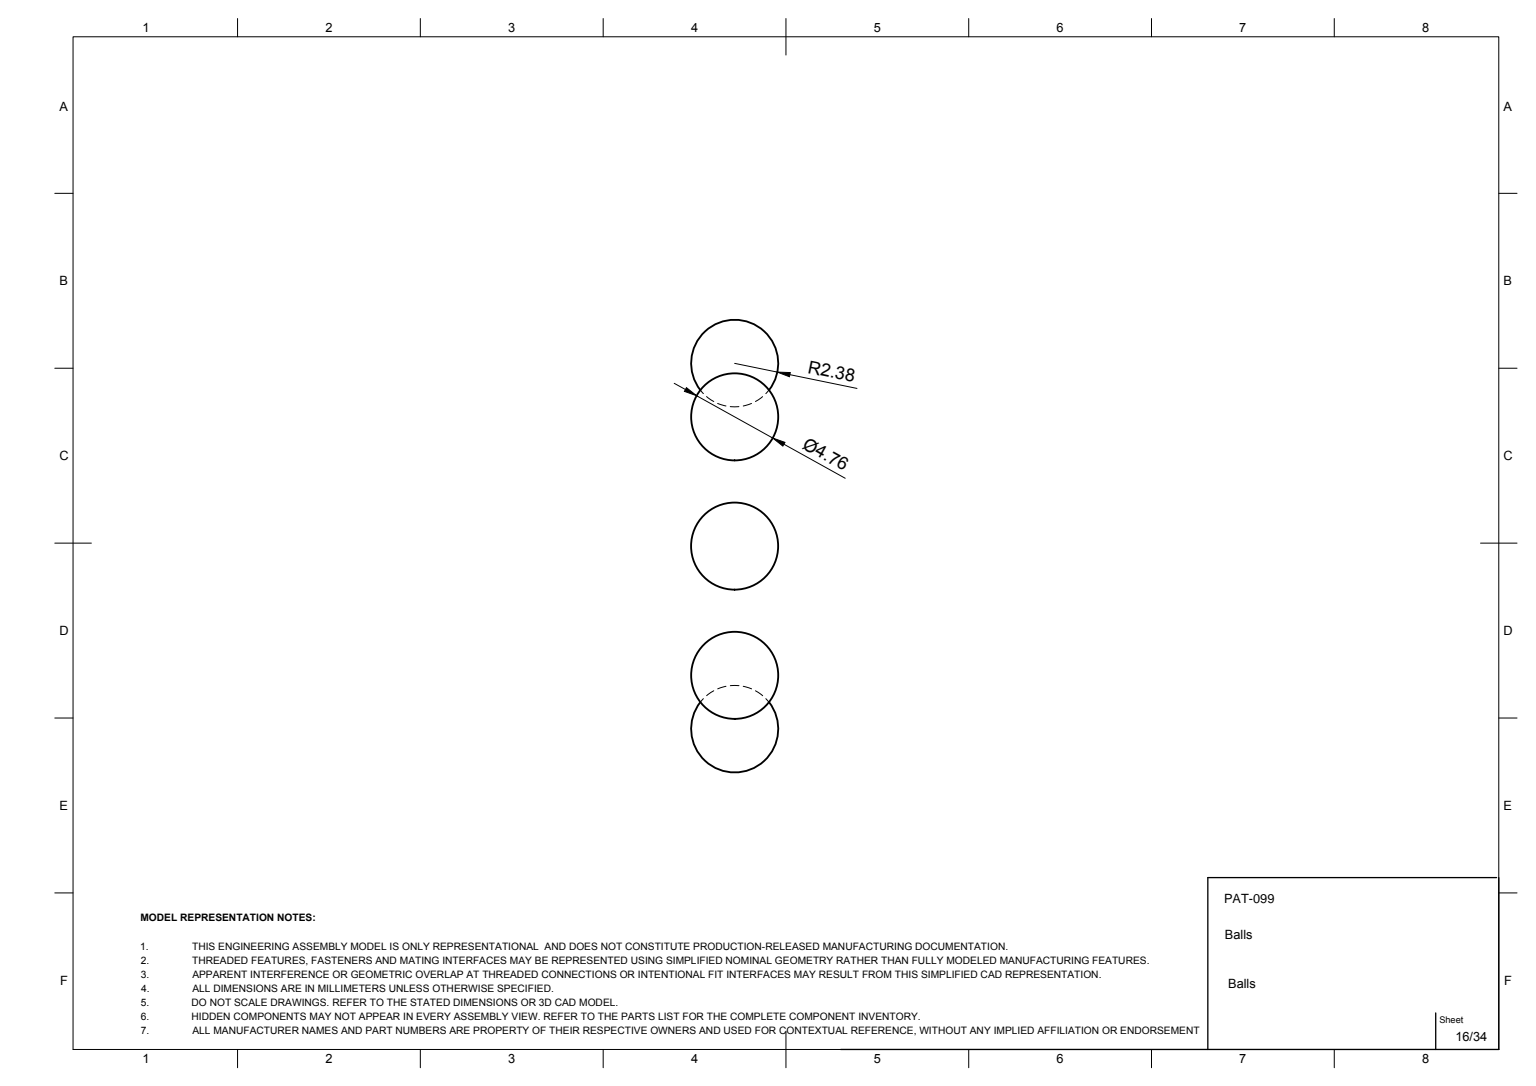
ISO-10303-21;
HEADER;
/* Generated by software containing ST-Developer
 * from STEP Tools, Inc. (www.steptools.com) 
 */

FILE_DESCRIPTION(
/* description */ ('PAT-099'),
/* implementation_level */ '2;1');

FILE_NAME(
/* name */ 'Balls.step',
/* time_stamp */ '2026-10-29T17:25:42-07:00',
/* author */ (''),
/* organization */ (''),
/* preprocessor_version */ 'ST-DEVELOPER v20.2',
/* originating_system */ 'Autodesk Translation Framework v15.17.0.0',
/* authorisation */ '');

FILE_SCHEMA (('AUTOMOTIVE_DESIGN { 1 0 10303 214 3 1 1 }'));
ENDSEC;

DATA;
#10=MECHANICAL_DESIGN_GEOMETRIC_PRESENTATION_REPRESENTATION('',(#359,#360,#361,#362,#363,#364,#365,#366),#11035);
#11=SPHERICAL_SURFACE('',#5544,0.23815);
#12=SPHERICAL_SURFACE('',#5546,0.23815);
#13=SPHERICAL_SURFACE('',#5548,0.23815);
#14=SPHERICAL_SURFACE('',#5550,0.23815);
#15=SPHERICAL_SURFACE('',#5552,0.23815);
#16=SPHERICAL_SURFACE('',#5554,0.23815);
#17=SPHERICAL_SURFACE('',#5556,0.23815);
#18=SPHERICAL_SURFACE('',#5558,0.23815);
#309=SHAPE_REPRESENTATION_RELATIONSHIP('SRR','None',#11182,#334);
#334=ADVANCED_BREP_SHAPE_REPRESENTATION('',(#390,#391,#392,#393,#394,#395,
#396,#397),#11032);
#359=STYLED_ITEM('',(#11386),#390);
#360=STYLED_ITEM('',(#11386),#391);
#361=STYLED_ITEM('',(#11386),#392);
#362=STYLED_ITEM('',(#11386),#393);
#363=STYLED_ITEM('',(#11386),#394);
#364=STYLED_ITEM('',(#11386),#395);
#365=STYLED_ITEM('',(#11386),#396);
#366=STYLED_ITEM('',(#11386),#397);
#390=MANIFOLD_SOLID_BREP('Body1',#4729);
#391=MANIFOLD_SOLID_BREP('Body2',#4730);
#392=MANIFOLD_SOLID_BREP('Body3',#4731);
#393=MANIFOLD_SOLID_BREP('Body4',#4732);
#394=MANIFOLD_SOLID_BREP('Body5',#4733);
#395=MANIFOLD_SOLID_BREP('Body6',#4734);
#396=MANIFOLD_SOLID_BREP('Body7',#4735);
#397=MANIFOLD_SOLID_BREP('Body8',#4736);
#905=FACE_OUTER_BOUND('',#1303,.T.);
#906=FACE_OUTER_BOUND('',#1304,.T.);
#907=FACE_OUTER_BOUND('',#1305,.T.);
#908=FACE_OUTER_BOUND('',#1306,.T.);
#909=FACE_OUTER_BOUND('',#1307,.T.);
#910=FACE_OUTER_BOUND('',#1308,.T.);
#911=FACE_OUTER_BOUND('',#1309,.T.);
#912=FACE_OUTER_BOUND('',#1310,.T.);
#1303=EDGE_LOOP('',(#4161,#4162));
#1304=EDGE_LOOP('',(#4163,#4164));
#1305=EDGE_LOOP('',(#4165,#4166));
#1306=EDGE_LOOP('',(#4167,#4168));
#1307=EDGE_LOOP('',(#4169,#4170));
#1308=EDGE_LOOP('',(#4171,#4172));
#1309=EDGE_LOOP('',(#4173,#4174));
#1310=EDGE_LOOP('',(#4175,#4176));
#2088=CIRCLE('',#5545,0.23815);
#2089=CIRCLE('',#5547,0.23815);
#2090=CIRCLE('',#5549,0.23815);
#2091=CIRCLE('',#5551,0.23815);
#2092=CIRCLE('',#5553,0.23815);
#2093=CIRCLE('',#5555,0.23815);
#2094=CIRCLE('',#5557,0.23815);
#2095=CIRCLE('',#5559,0.23815);
#2482=VERTEX_POINT('',#10425);
#2483=VERTEX_POINT('',#10426);
#2484=VERTEX_POINT('',#10429);
#2485=VERTEX_POINT('',#10430);
#2486=VERTEX_POINT('',#10433);
#2487=VERTEX_POINT('',#10434);
#2488=VERTEX_POINT('',#10437);
#2489=VERTEX_POINT('',#10438);
#2490=VERTEX_POINT('',#10441);
#2491=VERTEX_POINT('',#10442);
#2492=VERTEX_POINT('',#10445);
#2493=VERTEX_POINT('',#10446);
#2494=VERTEX_POINT('',#10449);
#2495=VERTEX_POINT('',#10450);
#2496=VERTEX_POINT('',#10453);
#2497=VERTEX_POINT('',#10454);
#3057=EDGE_CURVE('',#2482,#2483,#2088,.T.);
#3058=EDGE_CURVE('',#2484,#2485,#2089,.T.);
#3059=EDGE_CURVE('',#2486,#2487,#2090,.T.);
#3060=EDGE_CURVE('',#2488,#2489,#2091,.T.);
#3061=EDGE_CURVE('',#2490,#2491,#2092,.T.);
#3062=EDGE_CURVE('',#2492,#2493,#2093,.T.);
#3063=EDGE_CURVE('',#2494,#2495,#2094,.T.);
#3064=EDGE_CURVE('',#2496,#2497,#2095,.T.);
#4161=ORIENTED_EDGE('',*,*,#3057,.T.);
#4162=ORIENTED_EDGE('',*,*,#3057,.F.);
#4163=ORIENTED_EDGE('',*,*,#3058,.T.);
#4164=ORIENTED_EDGE('',*,*,#3058,.F.);
#4165=ORIENTED_EDGE('',*,*,#3059,.T.);
#4166=ORIENTED_EDGE('',*,*,#3059,.F.);
#4167=ORIENTED_EDGE('',*,*,#3060,.T.);
#4168=ORIENTED_EDGE('',*,*,#3060,.F.);
#4169=ORIENTED_EDGE('',*,*,#3061,.T.);
#4170=ORIENTED_EDGE('',*,*,#3061,.F.);
#4171=ORIENTED_EDGE('',*,*,#3062,.T.);
#4172=ORIENTED_EDGE('',*,*,#3062,.F.);
#4173=ORIENTED_EDGE('',*,*,#3063,.T.);
#4174=ORIENTED_EDGE('',*,*,#3063,.F.);
#4175=ORIENTED_EDGE('',*,*,#3064,.T.);
#4176=ORIENTED_EDGE('',*,*,#3064,.F.);
#4670=ADVANCED_FACE('',(#905),#11,.T.);
#4671=ADVANCED_FACE('',(#906),#12,.T.);
#4672=ADVANCED_FACE('',(#907),#13,.T.);
#4673=ADVANCED_FACE('',(#908),#14,.T.);
#4674=ADVANCED_FACE('',(#909),#15,.T.);
#4675=ADVANCED_FACE('',(#910),#16,.T.);
#4676=ADVANCED_FACE('',(#911),#17,.T.);
#4677=ADVANCED_FACE('',(#912),#18,.T.);
#4729=CLOSED_SHELL('',(#4670));
#4730=CLOSED_SHELL('',(#4671));
#4731=CLOSED_SHELL('',(#4672));
#4732=CLOSED_SHELL('',(#4673));
#4733=CLOSED_SHELL('',(#4674));
#4734=CLOSED_SHELL('',(#4675));
#4735=CLOSED_SHELL('',(#4676));
#4736=CLOSED_SHELL('',(#4677));
#5543=AXIS2_PLACEMENT_3D('',#10423,#6968,#6969);
#5544=AXIS2_PLACEMENT_3D('',#10424,#6970,#6971);
#5545=AXIS2_PLACEMENT_3D('',#10427,#6972,#6973);
#5546=AXIS2_PLACEMENT_3D('',#10428,#6974,#6975);
#5547=AXIS2_PLACEMENT_3D('',#10431,#6976,#6977);
#5548=AXIS2_PLACEMENT_3D('',#10432,#6978,#6979);
#5549=AXIS2_PLACEMENT_3D('',#10435,#6980,#6981);
#5550=AXIS2_PLACEMENT_3D('',#10436,#6982,#6983);
#5551=AXIS2_PLACEMENT_3D('',#10439,#6984,#6985);
#5552=AXIS2_PLACEMENT_3D('',#10440,#6986,#6987);
#5553=AXIS2_PLACEMENT_3D('',#10443,#6988,#6989);
#5554=AXIS2_PLACEMENT_3D('',#10444,#6990,#6991);
#5555=AXIS2_PLACEMENT_3D('',#10447,#6992,#6993);
#5556=AXIS2_PLACEMENT_3D('',#10448,#6994,#6995);
#5557=AXIS2_PLACEMENT_3D('',#10451,#6996,#6997);
#5558=AXIS2_PLACEMENT_3D('',#10452,#6998,#6999);
#5559=AXIS2_PLACEMENT_3D('',#10455,#7000,#7001);
#6968=DIRECTION('axis',(0.,0.,1.));
#6969=DIRECTION('refdir',(1.,0.,0.));
#6970=DIRECTION('center_axis',(0.,0.,1.));
#6971=DIRECTION('ref_axis',(1.,0.,0.));
#6972=DIRECTION('center_axis',(1.22464679914735E-16,-1.,0.));
#6973=DIRECTION('ref_axis',(-1.,-1.22464679914735E-16,0.));
#6974=DIRECTION('center_axis',(0.707106781186548,0.,0.707106781186548));
#6975=DIRECTION('ref_axis',(0.707106781186548,0.,-0.707106781186548));
#6976=DIRECTION('center_axis',(8.65956056235494E-17,-1.,-8.65956056235493E-17));
#6977=DIRECTION('ref_axis',(-0.707106781186547,-1.22464679914735E-16,0.707106781186547));
#6978=DIRECTION('center_axis',(1.,0.,0.));
#6979=DIRECTION('ref_axis',(6.12323399573676E-17,0.,-1.));
#6980=DIRECTION('center_axis',(7.49879891330929E-33,-1.,-1.22464679914735E-16));
#6981=DIRECTION('ref_axis',(-6.12323399573676E-17,-1.22464679914735E-16,
1.));
#6982=DIRECTION('center_axis',(0.707106781186548,0.,-0.707106781186548));
#6983=DIRECTION('ref_axis',(-0.707106781186548,0.,-0.707106781186548));
#6984=DIRECTION('center_axis',(-8.65956056235493E-17,-1.,-8.65956056235494E-17));
#6985=DIRECTION('ref_axis',(0.707106781186547,-1.22464679914735E-16,0.707106781186547));
#6986=DIRECTION('center_axis',(0.,0.,-1.));
#6987=DIRECTION('ref_axis',(-1.,0.,-1.22464679914735E-16));
#6988=DIRECTION('center_axis',(-1.22464679914735E-16,-1.,-1.49975978266186E-32));
#6989=DIRECTION('ref_axis',(1.,-1.22464679914735E-16,1.22464679914735E-16));
#6990=DIRECTION('center_axis',(-0.707106781186547,0.,-0.707106781186548));
#6991=DIRECTION('ref_axis',(-0.707106781186548,0.,0.707106781186547));
#6992=DIRECTION('center_axis',(-8.65956056235493E-17,-1.,8.65956056235493E-17));
#6993=DIRECTION('ref_axis',(0.707106781186548,-1.22464679914735E-16,-0.707106781186547));
#6994=DIRECTION('center_axis',(-1.,0.,0.));
#6995=DIRECTION('ref_axis',(-1.83697019872103E-16,0.,1.));
#6996=DIRECTION('center_axis',(-2.24963967399279E-32,-1.,1.22464679914735E-16));
#6997=DIRECTION('ref_axis',(1.83697019872103E-16,-1.22464679914735E-16,
-1.));
#6998=DIRECTION('center_axis',(-0.707106781186548,0.,0.707106781186548));
#6999=DIRECTION('ref_axis',(0.707106781186547,0.,0.707106781186548));
#7000=DIRECTION('center_axis',(8.65956056235493E-17,-1.,8.65956056235493E-17));
#7001=DIRECTION('ref_axis',(-0.707106781186547,-1.22464679914735E-16,-0.707106781186548));
#10423=CARTESIAN_POINT('',(0.,0.,0.));
#10424=CARTESIAN_POINT('Origin',(1.,0.,0.));
#10425=CARTESIAN_POINT('',(1.,-1.78583896120461E-33,0.23815));
#10426=CARTESIAN_POINT('',(1.,-1.78583896120461E-33,-0.23815));
#10427=CARTESIAN_POINT('Origin',(1.,0.,0.));
#10428=CARTESIAN_POINT('Origin',(0.707106781186548,0.,-0.707106781186547));
#10429=CARTESIAN_POINT('',(0.875504261126124,-1.78583896120461E-33,-0.538709301246971));
#10430=CARTESIAN_POINT('',(0.538709301246971,-1.78583896120461E-33,-0.875504261126124));
#10431=CARTESIAN_POINT('Origin',(0.707106781186548,0.,-0.707106781186547));
#10432=CARTESIAN_POINT('Origin',(6.12323399573677E-17,0.,-1.));
#10433=CARTESIAN_POINT('',(0.23815,-1.78583896120461E-33,-1.));
#10434=CARTESIAN_POINT('',(-0.23815,-1.78583896120461E-33,-1.));
#10435=CARTESIAN_POINT('Origin',(6.12323399573677E-17,0.,-1.));
#10436=CARTESIAN_POINT('Origin',(-0.707106781186547,0.,-0.707106781186548));
#10437=CARTESIAN_POINT('',(-0.538709301246971,-1.78583896120461E-33,-0.875504261126124));
#10438=CARTESIAN_POINT('',(-0.875504261126124,-1.78583896120461E-33,-0.538709301246971));
#10439=CARTESIAN_POINT('Origin',(-0.707106781186547,0.,-0.707106781186548));
#10440=CARTESIAN_POINT('Origin',(-1.,0.,-1.22464679914735E-16));
#10441=CARTESIAN_POINT('',(-1.,-1.78583896120461E-33,-0.23815));
#10442=CARTESIAN_POINT('',(-1.,-1.78583896120461E-33,0.23815));
#10443=CARTESIAN_POINT('Origin',(-1.,0.,-1.22464679914735E-16));
#10444=CARTESIAN_POINT('Origin',(-0.707106781186548,0.,0.707106781186547));
#10445=CARTESIAN_POINT('',(-0.875504261126124,-7.94881478324376E-33,0.538709301246971));
#10446=CARTESIAN_POINT('',(-0.538709301246971,4.37713686083455E-33,0.875504261126124));
#10447=CARTESIAN_POINT('Origin',(-0.707106781186548,0.,0.707106781186547));
#10448=CARTESIAN_POINT('Origin',(-1.83697019872103E-16,0.,1.));
#10449=CARTESIAN_POINT('',(-0.23815,-1.78583896120461E-33,1.));
#10450=CARTESIAN_POINT('',(0.23815,-1.78583896120461E-33,1.));
#10451=CARTESIAN_POINT('Origin',(-1.83697019872103E-16,0.,1.));
#10452=CARTESIAN_POINT('Origin',(0.707106781186547,0.,0.707106781186548));
#10453=CARTESIAN_POINT('',(0.538709301246971,-4.86732687222419E-33,0.875504261126124));
#10454=CARTESIAN_POINT('',(0.875504261126124,1.29564894981497E-33,0.538709301246971));
#10455=CARTESIAN_POINT('Origin',(0.707106781186547,0.,0.707106781186548));
#10999=UNCERTAINTY_MEASURE_WITH_UNIT(LENGTH_MEASURE(0.001),#11036,
'DISTANCE_ACCURACY_VALUE',
'Maximum model space distance between geometric entities at asserted c
onnectivities');
#11002=UNCERTAINTY_MEASURE_WITH_UNIT(LENGTH_MEASURE(0.001),#11036,
'DISTANCE_ACCURACY_VALUE',
'Maximum model space distance between geometric entities at asserted c
onnectivities');
#11032=(
GEOMETRIC_REPRESENTATION_CONTEXT(3)
GLOBAL_UNCERTAINTY_ASSIGNED_CONTEXT((#10999))
GLOBAL_UNIT_ASSIGNED_CONTEXT((#11036,#11038,#11039))
REPRESENTATION_CONTEXT('','3D')
);
#11035=(
GEOMETRIC_REPRESENTATION_CONTEXT(3)
GLOBAL_UNCERTAINTY_ASSIGNED_CONTEXT((#11002))
GLOBAL_UNIT_ASSIGNED_CONTEXT((#11036,#11038,#11039))
REPRESENTATION_CONTEXT('','3D')
);
#11036=(
LENGTH_UNIT()
NAMED_UNIT(*)
SI_UNIT(.CENTI.,.METRE.)
);
#11038=(
NAMED_UNIT(*)
PLANE_ANGLE_UNIT()
SI_UNIT($,.RADIAN.)
);
#11039=(
NAMED_UNIT(*)
SI_UNIT($,.STERADIAN.)
SOLID_ANGLE_UNIT()
);
#11069=SHAPE_DEFINITION_REPRESENTATION(#11113,#11182);
#11113=PRODUCT_DEFINITION_SHAPE('',$,#11215);
#11182=SHAPE_REPRESENTATION('',(#5543),#11032);
#11185=PRODUCT_DEFINITION_CONTEXT('part definition',#11283,'design');
#11215=PRODUCT_DEFINITION('Balls','Balls',#11247,#11185);
#11247=PRODUCT_DEFINITION_FORMATION('',$,#11314);
#11283=APPLICATION_CONTEXT(
'Core Data for Automotive Mechanical Design Process');
#11284=PRODUCT_CONTEXT('part definition',#11283,'mechanical');
#11314=PRODUCT('Balls','Balls','Balls',(#11284));
#11380=COLOUR_RGB('Grey',0.48,0.52,0.57);
#11381=FILL_AREA_STYLE_COLOUR('',#11380);
#11382=FILL_AREA_STYLE('',(#11381));
#11383=SURFACE_STYLE_FILL_AREA(#11382);
#11384=SURFACE_SIDE_STYLE('',(#11383));
#11385=SURFACE_STYLE_USAGE(.BOTH.,#11384);
#11386=PRESENTATION_STYLE_ASSIGNMENT((#11385));
ENDSEC;
END-ISO-10303-21;
